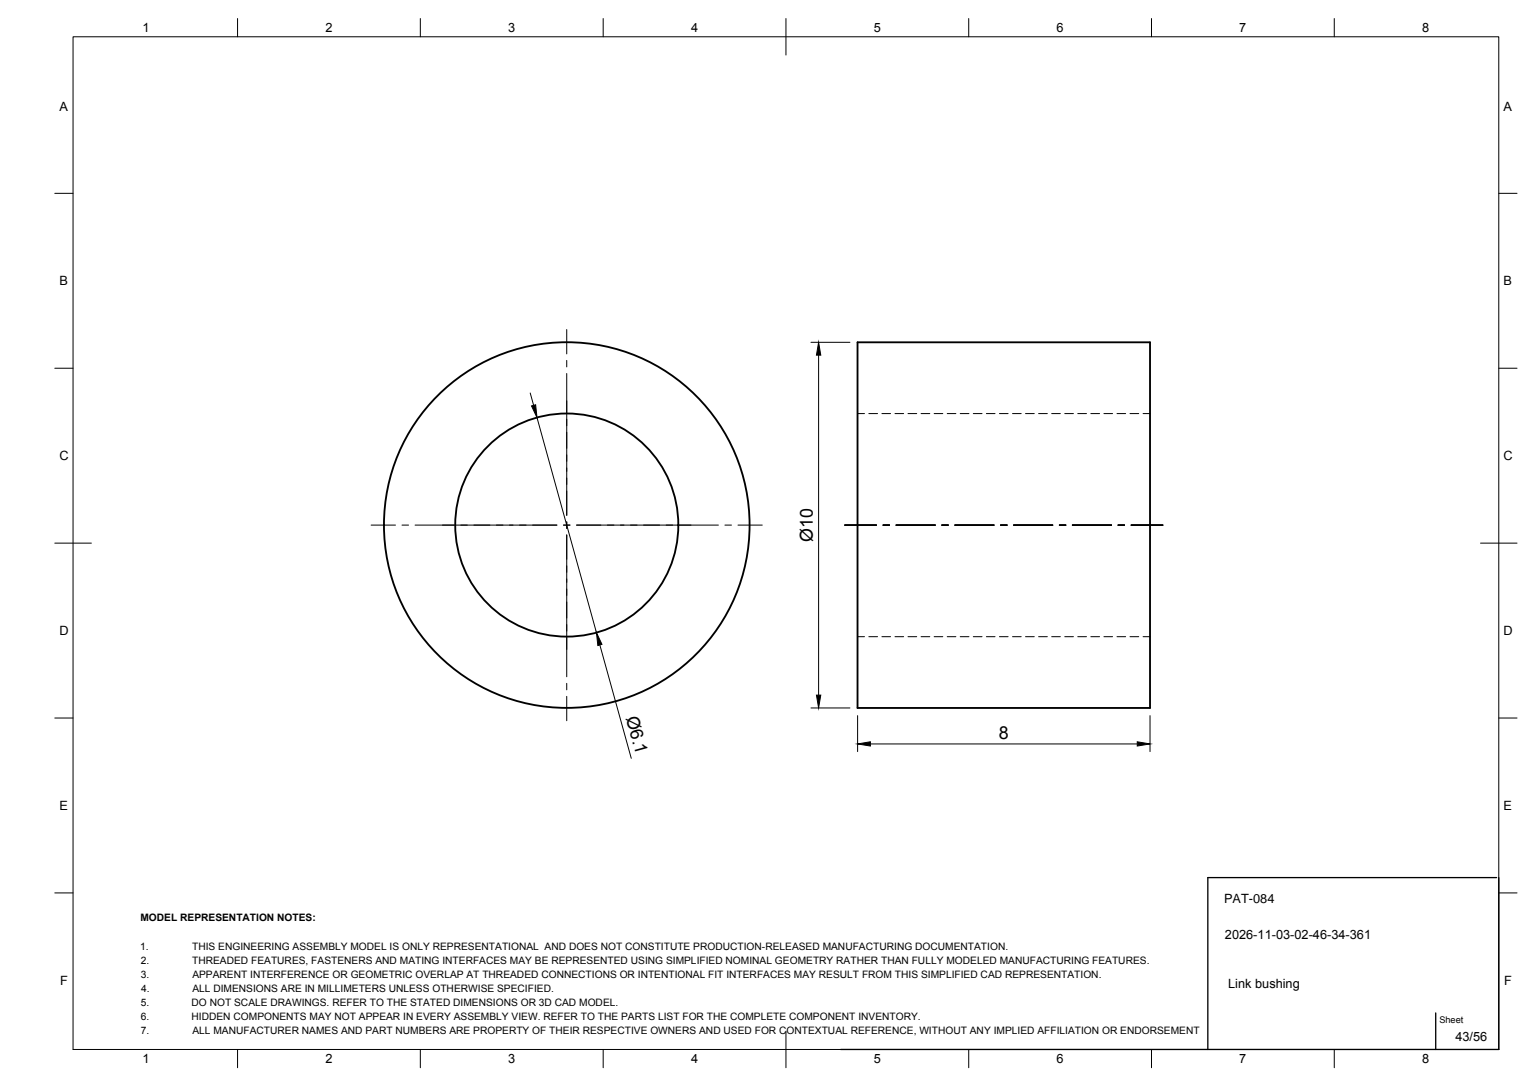
ISO-10303-21;
HEADER;
/* Generated by software containing ST-Developer
 * from STEP Tools, Inc. (www.steptools.com) 
 */

FILE_DESCRIPTION(
/* description */ ('Quick-return (Whitworth) mechanism'),
/* implementation_level */ '2;1');

FILE_NAME(
/* name */ 'Link bushing.step',
/* time_stamp */ '2026-10-28T03:25:57-07:00',
/* author */ (''),
/* organization */ (''),
/* preprocessor_version */ 'ST-DEVELOPER v20.2',
/* originating_system */ 'Autodesk Translation Framework v15.17.0.0',
/* authorisation */ '');

FILE_SCHEMA (('AUTOMOTIVE_DESIGN { 1 0 10303 214 3 1 1 }'));
ENDSEC;

DATA;
#10=MECHANICAL_DESIGN_GEOMETRIC_PRESENTATION_REPRESENTATION('',(#530),#14878);
#434=SHAPE_REPRESENTATION_RELATIONSHIP('SRR','None',#15107,#478);
#478=ADVANCED_BREP_SHAPE_REPRESENTATION('',(#581),#14864);
#530=STYLED_ITEM('',(#15392),#581);
#581=MANIFOLD_SOLID_BREP('Body1',#7885);
#753=FACE_BOUND('',#2030,.T.);
#754=FACE_BOUND('',#2032,.T.);
#966=PLANE('',#9135);
#967=PLANE('',#9136);
#1399=FACE_OUTER_BOUND('',#2027,.T.);
#1400=FACE_OUTER_BOUND('',#2028,.T.);
#1401=FACE_OUTER_BOUND('',#2029,.T.);
#1402=FACE_OUTER_BOUND('',#2031,.T.);
#2027=EDGE_LOOP('',(#6712,#6713,#6714,#6715));
#2028=EDGE_LOOP('',(#6716,#6717,#6718,#6719));
#2029=EDGE_LOOP('',(#6720));
#2030=EDGE_LOOP('',(#6721));
#2031=EDGE_LOOP('',(#6722));
#2032=EDGE_LOOP('',(#6723));
#2512=LINE('',#14162,#3035);
#2513=LINE('',#14168,#3036);
#3035=VECTOR('',#11233,0.305);
#3036=VECTOR('',#11240,0.5);
#3563=CIRCLE('',#9130,0.305);
#3564=CIRCLE('',#9131,0.305);
#3565=CIRCLE('',#9133,0.5);
#3566=CIRCLE('',#9134,0.5);
#4124=VERTEX_POINT('',#14159);
#4125=VERTEX_POINT('',#14161);
#4126=VERTEX_POINT('',#14165);
#4127=VERTEX_POINT('',#14167);
#5013=EDGE_CURVE('',#4124,#4124,#3563,.T.);
#5014=EDGE_CURVE('',#4124,#4125,#2512,.T.);
#5015=EDGE_CURVE('',#4125,#4125,#3564,.T.);
#5016=EDGE_CURVE('',#4126,#4126,#3565,.T.);
#5017=EDGE_CURVE('',#4126,#4127,#2513,.T.);
#5018=EDGE_CURVE('',#4127,#4127,#3566,.T.);
#6712=ORIENTED_EDGE('',*,*,#5013,.F.);
#6713=ORIENTED_EDGE('',*,*,#5014,.T.);
#6714=ORIENTED_EDGE('',*,*,#5015,.T.);
#6715=ORIENTED_EDGE('',*,*,#5014,.F.);
#6716=ORIENTED_EDGE('',*,*,#5016,.F.);
#6717=ORIENTED_EDGE('',*,*,#5017,.T.);
#6718=ORIENTED_EDGE('',*,*,#5018,.T.);
#6719=ORIENTED_EDGE('',*,*,#5017,.F.);
#6720=ORIENTED_EDGE('',*,*,#5016,.T.);
#6721=ORIENTED_EDGE('',*,*,#5013,.T.);
#6722=ORIENTED_EDGE('',*,*,#5018,.F.);
#6723=ORIENTED_EDGE('',*,*,#5015,.F.);
#7351=CYLINDRICAL_SURFACE('',#9129,0.305);
#7352=CYLINDRICAL_SURFACE('',#9132,0.5);
#7730=ADVANCED_FACE('',(#1399),#7351,.F.);
#7731=ADVANCED_FACE('',(#1400),#7352,.T.);
#7732=ADVANCED_FACE('',(#1401,#753),#966,.T.);
#7733=ADVANCED_FACE('',(#1402,#754),#967,.F.);
#7885=CLOSED_SHELL('',(#7730,#7731,#7732,#7733));
#9128=AXIS2_PLACEMENT_3D('',#14157,#11227,#11228);
#9129=AXIS2_PLACEMENT_3D('',#14158,#11229,#11230);
#9130=AXIS2_PLACEMENT_3D('',#14160,#11231,#11232);
#9131=AXIS2_PLACEMENT_3D('',#14163,#11234,#11235);
#9132=AXIS2_PLACEMENT_3D('',#14164,#11236,#11237);
#9133=AXIS2_PLACEMENT_3D('',#14166,#11238,#11239);
#9134=AXIS2_PLACEMENT_3D('',#14169,#11241,#11242);
#9135=AXIS2_PLACEMENT_3D('',#14170,#11243,#11244);
#9136=AXIS2_PLACEMENT_3D('',#14171,#11245,#11246);
#11227=DIRECTION('axis',(0.,0.,1.));
#11228=DIRECTION('refdir',(1.,0.,0.));
#11229=DIRECTION('center_axis',(0.,0.,1.));
#11230=DIRECTION('ref_axis',(1.,0.,0.));
#11231=DIRECTION('center_axis',(0.,0.,-1.));
#11232=DIRECTION('ref_axis',(1.,0.,0.));
#11233=DIRECTION('',(0.,0.,-1.));
#11234=DIRECTION('center_axis',(0.,0.,-1.));
#11235=DIRECTION('ref_axis',(1.,0.,0.));
#11236=DIRECTION('center_axis',(0.,0.,1.));
#11237=DIRECTION('ref_axis',(1.,0.,0.));
#11238=DIRECTION('center_axis',(0.,0.,1.));
#11239=DIRECTION('ref_axis',(1.,0.,0.));
#11240=DIRECTION('',(0.,0.,-1.));
#11241=DIRECTION('center_axis',(0.,0.,1.));
#11242=DIRECTION('ref_axis',(1.,0.,0.));
#11243=DIRECTION('center_axis',(0.,0.,1.));
#11244=DIRECTION('ref_axis',(1.,0.,0.));
#11245=DIRECTION('center_axis',(0.,0.,1.));
#11246=DIRECTION('ref_axis',(1.,0.,0.));
#14157=CARTESIAN_POINT('',(0.,0.,0.));
#14158=CARTESIAN_POINT('Origin',(0.,12.,8.4));
#14159=CARTESIAN_POINT('',(-0.305,12.,9.2));
#14160=CARTESIAN_POINT('Origin',(0.,12.,9.2));
#14161=CARTESIAN_POINT('',(-0.305,12.,8.4));
#14162=CARTESIAN_POINT('',(-0.305,12.,8.4));
#14163=CARTESIAN_POINT('Origin',(0.,12.,8.4));
#14164=CARTESIAN_POINT('Origin',(0.,12.,8.4));
#14165=CARTESIAN_POINT('',(-0.5,12.,9.2));
#14166=CARTESIAN_POINT('Origin',(0.,12.,9.2));
#14167=CARTESIAN_POINT('',(-0.5,12.,8.4));
#14168=CARTESIAN_POINT('',(-0.5,12.,8.4));
#14169=CARTESIAN_POINT('Origin',(0.,12.,8.4));
#14170=CARTESIAN_POINT('Origin',(0.,12.,9.2));
#14171=CARTESIAN_POINT('Origin',(0.,12.,8.4));
#14810=UNCERTAINTY_MEASURE_WITH_UNIT(LENGTH_MEASURE(0.001),#14879,
'DISTANCE_ACCURACY_VALUE',
'Maximum model space distance between geometric entities at asserted c
onnectivities');
#14824=UNCERTAINTY_MEASURE_WITH_UNIT(LENGTH_MEASURE(0.001),#14879,
'DISTANCE_ACCURACY_VALUE',
'Maximum model space distance between geometric entities at asserted c
onnectivities');
#14864=(
GEOMETRIC_REPRESENTATION_CONTEXT(3)
GLOBAL_UNCERTAINTY_ASSIGNED_CONTEXT((#14810))
GLOBAL_UNIT_ASSIGNED_CONTEXT((#14879,#14881,#14882))
REPRESENTATION_CONTEXT('','3D')
);
#14878=(
GEOMETRIC_REPRESENTATION_CONTEXT(3)
GLOBAL_UNCERTAINTY_ASSIGNED_CONTEXT((#14824))
GLOBAL_UNIT_ASSIGNED_CONTEXT((#14879,#14881,#14882))
REPRESENTATION_CONTEXT('','3D')
);
#14879=(
LENGTH_UNIT()
NAMED_UNIT(*)
SI_UNIT(.CENTI.,.METRE.)
);
#14881=(
NAMED_UNIT(*)
PLANE_ANGLE_UNIT()
SI_UNIT($,.RADIAN.)
);
#14882=(
NAMED_UNIT(*)
SI_UNIT($,.STERADIAN.)
SOLID_ANGLE_UNIT()
);
#14922=SHAPE_DEFINITION_REPRESENTATION(#14981,#15107);
#14981=PRODUCT_DEFINITION_SHAPE('',$,#15161);
#15107=SHAPE_REPRESENTATION('',(#9128),#14864);
#15121=PRODUCT_DEFINITION_CONTEXT('part definition',#15282,'design');
#15161=PRODUCT_DEFINITION('Link bushing','Link bushing',#15214,#15121);
#15214=PRODUCT_DEFINITION_FORMATION('',$,#15323);
#15282=APPLICATION_CONTEXT(
'Core Data for Automotive Mechanical Design Process');
#15283=PRODUCT_CONTEXT('part definition',#15282,'mechanical');
#15323=PRODUCT('Link bushing','Link bushing','Link bushing',(#15283));
#15386=COLOUR_RGB('Light Blue',0.38,0.62,0.78);
#15387=FILL_AREA_STYLE_COLOUR('',#15386);
#15388=FILL_AREA_STYLE('',(#15387));
#15389=SURFACE_STYLE_FILL_AREA(#15388);
#15390=SURFACE_SIDE_STYLE('',(#15389));
#15391=SURFACE_STYLE_USAGE(.BOTH.,#15390);
#15392=PRESENTATION_STYLE_ASSIGNMENT((#15391));
ENDSEC;
END-ISO-10303-21;
